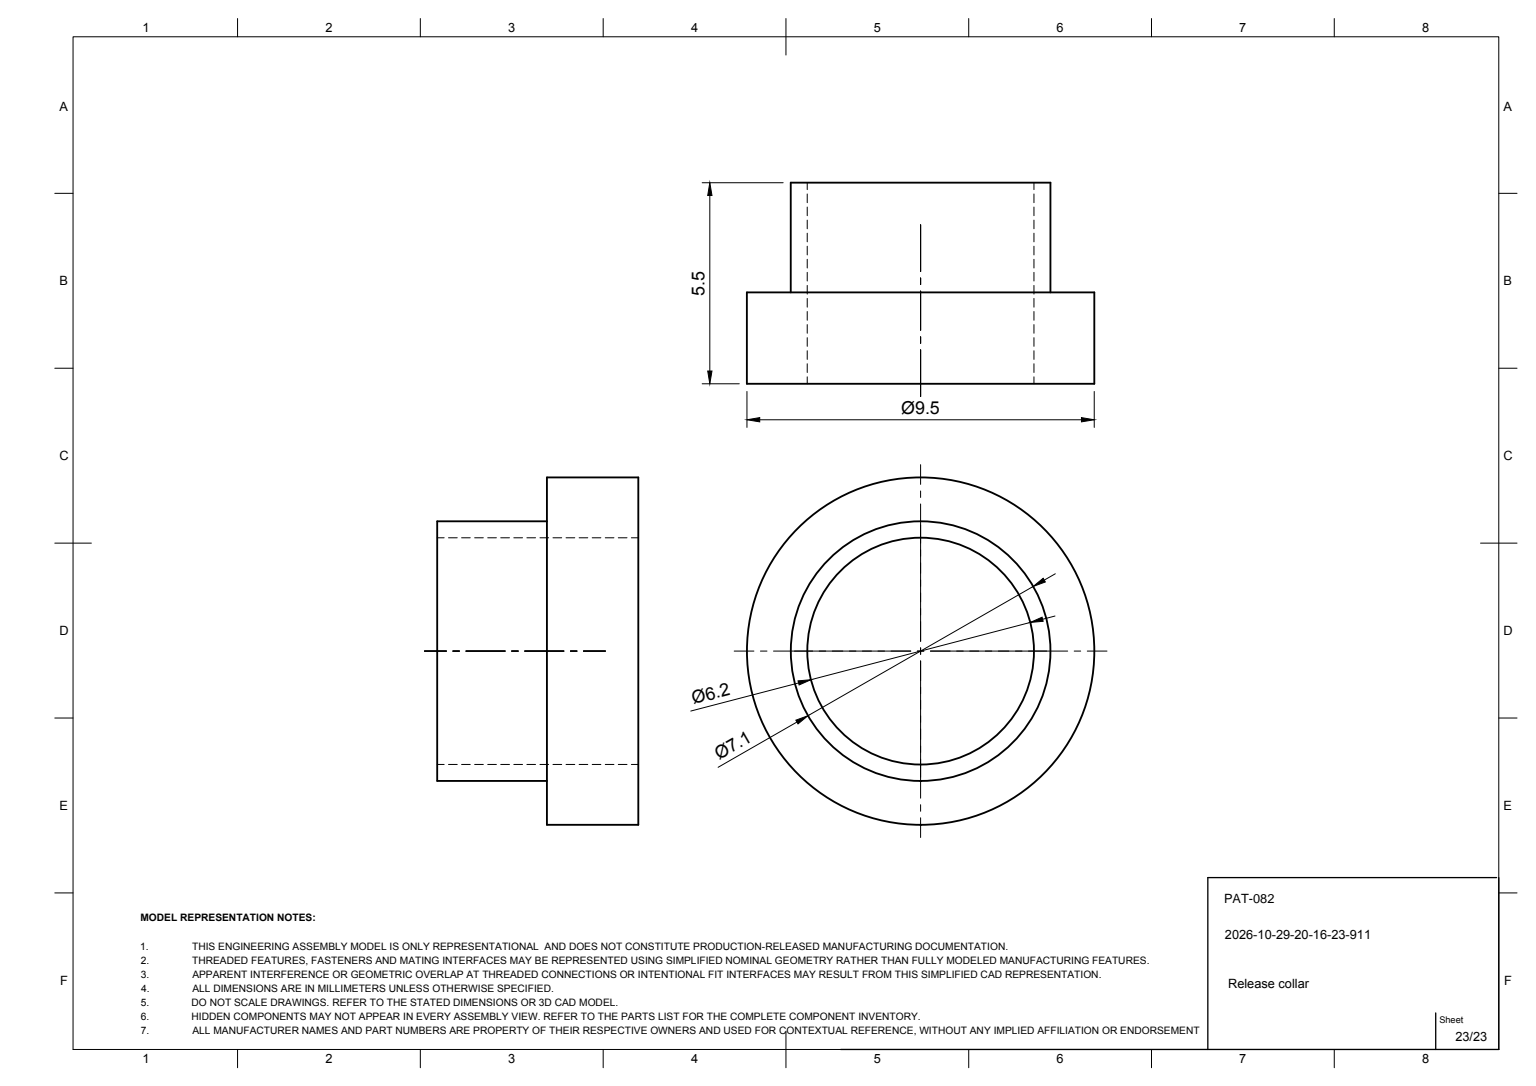
ISO-10303-21;
HEADER;
/* Generated by software containing ST-Developer
 * from STEP Tools, Inc. (www.steptools.com) 
 */

FILE_DESCRIPTION(
/* description */ ('PAT-082'),
/* implementation_level */ '2;1');

FILE_NAME(
/* name */ 'Release collar.step',
/* time_stamp */ '2026-10-29T20:16:13-07:00',
/* author */ (''),
/* organization */ (''),
/* preprocessor_version */ 'ST-DEVELOPER v20.2',
/* originating_system */ 'Autodesk Translation Framework v15.17.0.0',
/* authorisation */ '');

FILE_SCHEMA (('AUTOMOTIVE_DESIGN { 1 0 10303 214 3 1 1 }'));
ENDSEC;

DATA;
#10=MECHANICAL_DESIGN_GEOMETRIC_PRESENTATION_REPRESENTATION('',(#259),#8266);
#215=SHAPE_REPRESENTATION_RELATIONSHIP('SRR','None',#8378,#237);
#237=ADVANCED_BREP_SHAPE_REPRESENTATION('',(#280),#8262);
#259=STYLED_ITEM('',(#8551),#280);
#280=MANIFOLD_SOLID_BREP('Body1',#4600);
#396=FACE_BOUND('',#1173,.T.);
#397=FACE_BOUND('',#1176,.T.);
#398=FACE_BOUND('',#1179,.T.);
#537=PLANE('',#5257);
#538=PLANE('',#5262);
#539=PLANE('',#5266);
#788=FACE_OUTER_BOUND('',#1172,.T.);
#789=FACE_OUTER_BOUND('',#1174,.T.);
#790=FACE_OUTER_BOUND('',#1175,.T.);
#791=FACE_OUTER_BOUND('',#1177,.T.);
#792=FACE_OUTER_BOUND('',#1178,.T.);
#793=FACE_OUTER_BOUND('',#1180,.T.);
#1172=EDGE_LOOP('',(#4016));
#1173=EDGE_LOOP('',(#4017));
#1174=EDGE_LOOP('',(#4018,#4019,#4020,#4021));
#1175=EDGE_LOOP('',(#4022));
#1176=EDGE_LOOP('',(#4023));
#1177=EDGE_LOOP('',(#4024,#4025,#4026,#4027));
#1178=EDGE_LOOP('',(#4028));
#1179=EDGE_LOOP('',(#4029));
#1180=EDGE_LOOP('',(#4030,#4031,#4032,#4033));
#1517=LINE('',#7962,#1872);
#1518=LINE('',#7969,#1873);
#1519=LINE('',#7974,#1874);
#1872=VECTOR('',#6490,0.475);
#1873=VECTOR('',#6499,0.355);
#1874=VECTOR('',#6506,0.31);
#2116=CIRCLE('',#5258,0.475);
#2117=CIRCLE('',#5259,0.31);
#2118=CIRCLE('',#5261,0.475);
#2119=CIRCLE('',#5263,0.355);
#2120=CIRCLE('',#5265,0.355);
#2121=CIRCLE('',#5267,0.31);
#2454=VERTEX_POINT('',#7955);
#2455=VERTEX_POINT('',#7957);
#2456=VERTEX_POINT('',#7960);
#2457=VERTEX_POINT('',#7964);
#2458=VERTEX_POINT('',#7967);
#2459=VERTEX_POINT('',#7971);
#2984=EDGE_CURVE('',#2454,#2454,#2116,.T.);
#2985=EDGE_CURVE('',#2455,#2455,#2117,.T.);
#2986=EDGE_CURVE('',#2456,#2456,#2118,.T.);
#2987=EDGE_CURVE('',#2456,#2454,#1517,.T.);
#2988=EDGE_CURVE('',#2457,#2457,#2119,.T.);
#2989=EDGE_CURVE('',#2458,#2458,#2120,.T.);
#2990=EDGE_CURVE('',#2458,#2457,#1518,.T.);
#2991=EDGE_CURVE('',#2459,#2459,#2121,.T.);
#2992=EDGE_CURVE('',#2459,#2455,#1519,.T.);
#4016=ORIENTED_EDGE('',*,*,#2984,.F.);
#4017=ORIENTED_EDGE('',*,*,#2985,.T.);
#4018=ORIENTED_EDGE('',*,*,#2986,.F.);
#4019=ORIENTED_EDGE('',*,*,#2987,.T.);
#4020=ORIENTED_EDGE('',*,*,#2984,.T.);
#4021=ORIENTED_EDGE('',*,*,#2987,.F.);
#4022=ORIENTED_EDGE('',*,*,#2986,.T.);
#4023=ORIENTED_EDGE('',*,*,#2988,.F.);
#4024=ORIENTED_EDGE('',*,*,#2989,.F.);
#4025=ORIENTED_EDGE('',*,*,#2990,.T.);
#4026=ORIENTED_EDGE('',*,*,#2988,.T.);
#4027=ORIENTED_EDGE('',*,*,#2990,.F.);
#4028=ORIENTED_EDGE('',*,*,#2989,.T.);
#4029=ORIENTED_EDGE('',*,*,#2991,.F.);
#4030=ORIENTED_EDGE('',*,*,#2991,.T.);
#4031=ORIENTED_EDGE('',*,*,#2992,.T.);
#4032=ORIENTED_EDGE('',*,*,#2985,.F.);
#4033=ORIENTED_EDGE('',*,*,#2992,.F.);
#4301=CYLINDRICAL_SURFACE('',#5260,0.475);
#4302=CYLINDRICAL_SURFACE('',#5264,0.355);
#4303=CYLINDRICAL_SURFACE('',#5268,0.31);
#4527=ADVANCED_FACE('',(#788,#396),#537,.T.);
#4528=ADVANCED_FACE('',(#789),#4301,.T.);
#4529=ADVANCED_FACE('',(#790,#397),#538,.T.);
#4530=ADVANCED_FACE('',(#791),#4302,.T.);
#4531=ADVANCED_FACE('',(#792,#398),#539,.T.);
#4532=ADVANCED_FACE('',(#793),#4303,.F.);
#4600=CLOSED_SHELL('',(#4527,#4528,#4529,#4530,#4531,#4532));
#5256=AXIS2_PLACEMENT_3D('',#7953,#6478,#6479);
#5257=AXIS2_PLACEMENT_3D('',#7954,#6480,#6481);
#5258=AXIS2_PLACEMENT_3D('',#7956,#6482,#6483);
#5259=AXIS2_PLACEMENT_3D('',#7958,#6484,#6485);
#5260=AXIS2_PLACEMENT_3D('',#7959,#6486,#6487);
#5261=AXIS2_PLACEMENT_3D('',#7961,#6488,#6489);
#5262=AXIS2_PLACEMENT_3D('',#7963,#6491,#6492);
#5263=AXIS2_PLACEMENT_3D('',#7965,#6493,#6494);
#5264=AXIS2_PLACEMENT_3D('',#7966,#6495,#6496);
#5265=AXIS2_PLACEMENT_3D('',#7968,#6497,#6498);
#5266=AXIS2_PLACEMENT_3D('',#7970,#6500,#6501);
#5267=AXIS2_PLACEMENT_3D('',#7972,#6502,#6503);
#5268=AXIS2_PLACEMENT_3D('',#7973,#6504,#6505);
#6478=DIRECTION('axis',(0.,0.,1.));
#6479=DIRECTION('refdir',(1.,0.,0.));
#6480=DIRECTION('center_axis',(0.,1.,0.));
#6481=DIRECTION('ref_axis',(0.,0.,1.));
#6482=DIRECTION('center_axis',(0.,-1.,0.));
#6483=DIRECTION('ref_axis',(1.,0.,0.));
#6484=DIRECTION('center_axis',(0.,-1.,0.));
#6485=DIRECTION('ref_axis',(1.,0.,0.));
#6486=DIRECTION('center_axis',(0.,-1.,0.));
#6487=DIRECTION('ref_axis',(1.,0.,0.));
#6488=DIRECTION('center_axis',(0.,-1.,0.));
#6489=DIRECTION('ref_axis',(1.,0.,0.));
#6490=DIRECTION('',(0.,1.,0.));
#6491=DIRECTION('center_axis',(0.,-1.,0.));
#6492=DIRECTION('ref_axis',(0.,0.,-1.));
#6493=DIRECTION('center_axis',(0.,-1.,0.));
#6494=DIRECTION('ref_axis',(1.,0.,0.));
#6495=DIRECTION('center_axis',(0.,-1.,0.));
#6496=DIRECTION('ref_axis',(1.,0.,0.));
#6497=DIRECTION('center_axis',(0.,-1.,0.));
#6498=DIRECTION('ref_axis',(1.,0.,0.));
#6499=DIRECTION('',(0.,1.,0.));
#6500=DIRECTION('center_axis',(0.,-1.,0.));
#6501=DIRECTION('ref_axis',(0.,0.,-1.));
#6502=DIRECTION('center_axis',(0.,-1.,0.));
#6503=DIRECTION('ref_axis',(1.,0.,0.));
#6504=DIRECTION('center_axis',(0.,-1.,0.));
#6505=DIRECTION('ref_axis',(1.,0.,0.));
#6506=DIRECTION('',(0.,1.,0.));
#7953=CARTESIAN_POINT('',(0.,0.,0.));
#7954=CARTESIAN_POINT('Origin',(0.475,1.95,0.));
#7955=CARTESIAN_POINT('',(-0.475,1.95,-5.81707229594993E-17));
#7956=CARTESIAN_POINT('Origin',(0.,1.95,0.));
#7957=CARTESIAN_POINT('',(-0.31,1.95,-3.7964050773568E-17));
#7958=CARTESIAN_POINT('Origin',(0.,1.95,0.));
#7959=CARTESIAN_POINT('Origin',(0.,1.825,0.));
#7960=CARTESIAN_POINT('',(-0.475,1.7,-5.81707229594993E-17));
#7961=CARTESIAN_POINT('Origin',(0.,1.7,0.));
#7962=CARTESIAN_POINT('',(-0.475,1.825,-5.81707229594993E-17));
#7963=CARTESIAN_POINT('Origin',(0.355,1.7,0.));
#7964=CARTESIAN_POINT('',(-0.355,1.7,-4.3474961369731E-17));
#7965=CARTESIAN_POINT('Origin',(0.,1.7,0.));
#7966=CARTESIAN_POINT('Origin',(0.,1.55,0.));
#7967=CARTESIAN_POINT('',(-0.355,1.4,-4.3474961369731E-17));
#7968=CARTESIAN_POINT('Origin',(0.,1.4,0.));
#7969=CARTESIAN_POINT('',(-0.355,1.55,-4.3474961369731E-17));
#7970=CARTESIAN_POINT('Origin',(0.31,1.4,0.));
#7971=CARTESIAN_POINT('',(-0.31,1.4,-3.7964050773568E-17));
#7972=CARTESIAN_POINT('Origin',(0.,1.4,0.));
#7973=CARTESIAN_POINT('Origin',(0.,1.675,0.));
#7974=CARTESIAN_POINT('',(-0.31,1.675,-3.7964050773568E-17));
#8237=UNCERTAINTY_MEASURE_WITH_UNIT(LENGTH_MEASURE(0.001),#8267,
'DISTANCE_ACCURACY_VALUE',
'Maximum model space distance between geometric entities at asserted c
onnectivities');
#8241=UNCERTAINTY_MEASURE_WITH_UNIT(LENGTH_MEASURE(0.001),#8267,
'DISTANCE_ACCURACY_VALUE',
'Maximum model space distance between geometric entities at asserted c
onnectivities');
#8262=(
GEOMETRIC_REPRESENTATION_CONTEXT(3)
GLOBAL_UNCERTAINTY_ASSIGNED_CONTEXT((#8237))
GLOBAL_UNIT_ASSIGNED_CONTEXT((#8267,#8269,#8270))
REPRESENTATION_CONTEXT('','3D')
);
#8266=(
GEOMETRIC_REPRESENTATION_CONTEXT(3)
GLOBAL_UNCERTAINTY_ASSIGNED_CONTEXT((#8241))
GLOBAL_UNIT_ASSIGNED_CONTEXT((#8267,#8269,#8270))
REPRESENTATION_CONTEXT('','3D')
);
#8267=(
LENGTH_UNIT()
NAMED_UNIT(*)
SI_UNIT(.CENTI.,.METRE.)
);
#8269=(
NAMED_UNIT(*)
PLANE_ANGLE_UNIT()
SI_UNIT($,.RADIAN.)
);
#8270=(
NAMED_UNIT(*)
SI_UNIT($,.STERADIAN.)
SOLID_ANGLE_UNIT()
);
#8291=SHAPE_DEFINITION_REPRESENTATION(#8315,#8378);
#8315=PRODUCT_DEFINITION_SHAPE('',$,#8403);
#8378=SHAPE_REPRESENTATION('',(#5256),#8262);
#8382=PRODUCT_DEFINITION_CONTEXT('part definition',#8456,'design');
#8403=PRODUCT_DEFINITION('Release collar','Release collar',#8427,
#8382);
#8427=PRODUCT_DEFINITION_FORMATION('',$,#8478);
#8456=APPLICATION_CONTEXT(
'Core Data for Automotive Mechanical Design Process');
#8457=PRODUCT_CONTEXT('part definition',#8456,'mechanical');
#8478=PRODUCT('Release collar','Release collar',
'Release collar',(#8457));
#8545=COLOUR_RGB('Off White',0.89,0.88,0.83);
#8546=FILL_AREA_STYLE_COLOUR('',#8545);
#8547=FILL_AREA_STYLE('',(#8546));
#8548=SURFACE_STYLE_FILL_AREA(#8547);
#8549=SURFACE_SIDE_STYLE('',(#8548));
#8550=SURFACE_STYLE_USAGE(.BOTH.,#8549);
#8551=PRESENTATION_STYLE_ASSIGNMENT((#8550));
ENDSEC;
END-ISO-10303-21;
